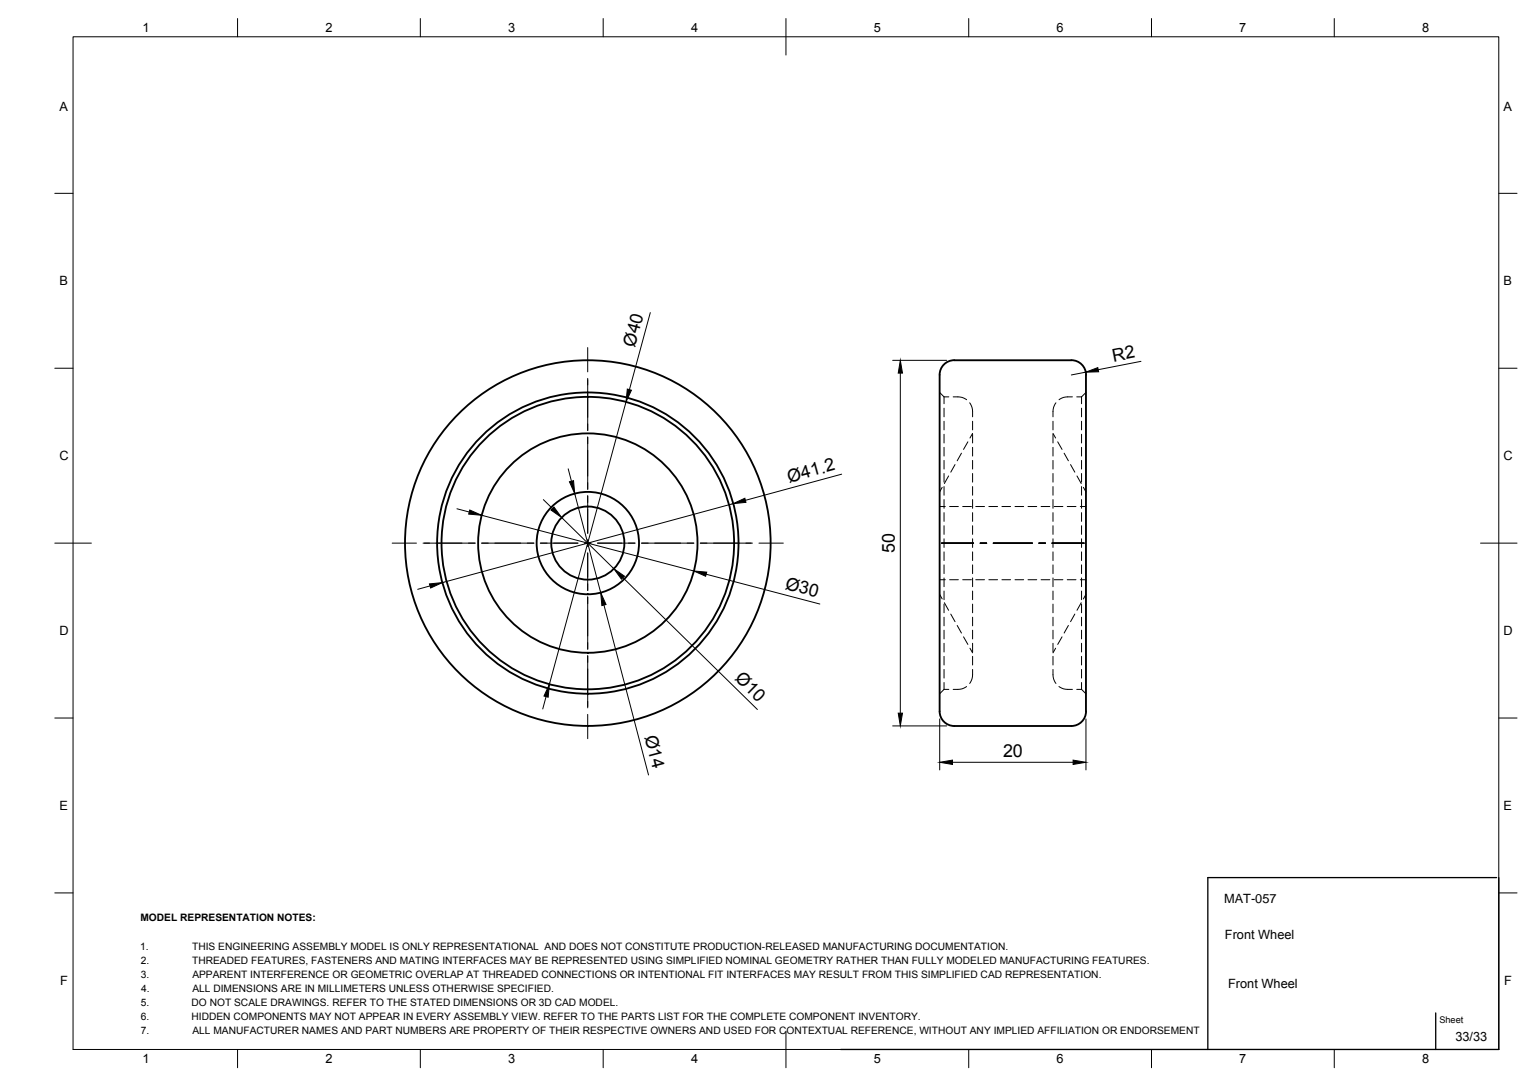
ISO-10303-21;
HEADER;
/* Generated by software containing ST-Developer
 * from STEP Tools, Inc. (www.steptools.com) 
 */

FILE_DESCRIPTION(
/* description */ ('STEP AP214', 'CAx-IF Rec.Pracs.---Representation and Presentation of Product Manufa
cturing Information (PMI)---4.0---2014-10-13'),
/* implementation_level */ '2;1');

FILE_NAME(
/* name */ 'Front Wheel.step',
/* time_stamp */ '2026-10-28T23:34:22+01:00',
/* author */ (''),
/* organization */ (''),
/* preprocessor_version */ 'ST-DEVELOPER v20.2',
/* originating_system */ 'Autodesk Translation Framework v15.17.0.0',
/* authorisation */ '');

FILE_SCHEMA (('AP242_MANAGED_MODEL_BASED_3D_ENGINEERING_MIM_LF { 1 0 10303 442 2 1 4 }'));
ENDSEC;

DATA;
#10=MECHANICAL_DESIGN_GEOMETRIC_PRESENTATION_REPRESENTATION('',(#272),#27807);
#224=SHAPE_REPRESENTATION_RELATIONSHIP('SRR','None',#27923,#246);
#246=ADVANCED_BREP_SHAPE_REPRESENTATION('',(#301),#27803);
#272=STYLED_ITEM('',(#28070),#301);
#301=MANIFOLD_SOLID_BREP('Body1',#12048);
#427=FACE_BOUND('',#2600,.T.);
#428=FACE_BOUND('',#2602,.T.);
#429=FACE_BOUND('',#2604,.T.);
#430=FACE_BOUND('',#2606,.T.);
#431=FACE_BOUND('',#2608,.T.);
#432=FACE_BOUND('',#2610,.T.);
#695=PLANE('',#13506);
#696=PLANE('',#13507);
#697=PLANE('',#13508);
#698=PLANE('',#13509);
#699=PLANE('',#13510);
#700=PLANE('',#13511);
#842=TOROIDAL_SURFACE('',#13475,23.,2.);
#843=TOROIDAL_SURFACE('',#13480,18.,2.);
#844=TOROIDAL_SURFACE('',#13484,23.,2.);
#845=TOROIDAL_SURFACE('',#13489,18.,2.);
#1180=CYLINDRICAL_SURFACE('',#13494,5.00000000000002);
#1181=CYLINDRICAL_SURFACE('',#13500,20.);
#1182=CYLINDRICAL_SURFACE('',#13504,20.);
#1183=CYLINDRICAL_SURFACE('',#13505,25.);
#1798=FACE_OUTER_BOUND('',#2587,.T.);
#1799=FACE_OUTER_BOUND('',#2588,.T.);
#1800=FACE_OUTER_BOUND('',#2589,.T.);
#1801=FACE_OUTER_BOUND('',#2590,.T.);
#1802=FACE_OUTER_BOUND('',#2591,.T.);
#1803=FACE_OUTER_BOUND('',#2592,.T.);
#1804=FACE_OUTER_BOUND('',#2593,.T.);
#1805=FACE_OUTER_BOUND('',#2594,.T.);
#1806=FACE_OUTER_BOUND('',#2595,.T.);
#1807=FACE_OUTER_BOUND('',#2596,.T.);
#1808=FACE_OUTER_BOUND('',#2597,.T.);
#1809=FACE_OUTER_BOUND('',#2598,.T.);
#1810=FACE_OUTER_BOUND('',#2599,.T.);
#1811=FACE_OUTER_BOUND('',#2601,.T.);
#1812=FACE_OUTER_BOUND('',#2603,.T.);
#1813=FACE_OUTER_BOUND('',#2605,.T.);
#1814=FACE_OUTER_BOUND('',#2607,.T.);
#1815=FACE_OUTER_BOUND('',#2609,.T.);
#2587=EDGE_LOOP('',(#10579,#10580,#10581,#10582,#10583));
#2588=EDGE_LOOP('',(#10584,#10585,#10586,#10587));
#2589=EDGE_LOOP('',(#10588,#10589,#10590,#10591,#10592));
#2590=EDGE_LOOP('',(#10593,#10594,#10595,#10596));
#2591=EDGE_LOOP('',(#10597,#10598,#10599,#10600,#10601));
#2592=EDGE_LOOP('',(#10602,#10603,#10604,#10605,#10606));
#2593=EDGE_LOOP('',(#10607,#10608,#10609,#10610));
#2594=EDGE_LOOP('',(#10611,#10612,#10613,#10614));
#2595=EDGE_LOOP('',(#10615,#10616,#10617,#10618));
#2596=EDGE_LOOP('',(#10619,#10620,#10621,#10622));
#2597=EDGE_LOOP('',(#10623,#10624,#10625,#10626,#10627,#10628));
#2598=EDGE_LOOP('',(#10629,#10630,#10631,#10632,#10633,#10634));
#2599=EDGE_LOOP('',(#10635));
#2600=EDGE_LOOP('',(#10636));
#2601=EDGE_LOOP('',(#10637));
#2602=EDGE_LOOP('',(#10638));
#2603=EDGE_LOOP('',(#10639));
#2604=EDGE_LOOP('',(#10640));
#2605=EDGE_LOOP('',(#10641));
#2606=EDGE_LOOP('',(#10642));
#2607=EDGE_LOOP('',(#10643));
#2608=EDGE_LOOP('',(#10644));
#2609=EDGE_LOOP('',(#10645));
#2610=EDGE_LOOP('',(#10646));
#3425=LINE('',#23241,#4245);
#3426=LINE('',#23247,#4246);
#3427=LINE('',#23283,#4247);
#3428=LINE('',#23289,#4248);
#3429=LINE('',#23292,#4249);
#3430=LINE('',#23297,#4250);
#3431=LINE('',#23300,#4251);
#3432=LINE('',#23302,#4252);
#4245=VECTOR('',#16749,20.6);
#4246=VECTOR('',#16756,20.);
#4247=VECTOR('',#16801,5.00000000000002);
#4248=VECTOR('',#16808,7.00000000000002);
#4249=VECTOR('',#16813,20.);
#4250=VECTOR('',#16818,15.);
#4251=VECTOR('',#16823,20.);
#4252=VECTOR('',#16826,25.);
#4940=CIRCLE('',#13469,20.);
#4941=CIRCLE('',#13470,20.);
#4942=CIRCLE('',#13471,20.6);
#4943=CIRCLE('',#13473,20.);
#4944=CIRCLE('',#13474,20.6);
#4945=CIRCLE('',#13476,23.);
#4946=CIRCLE('',#13477,2.);
#4947=CIRCLE('',#13478,25.);
#4948=CIRCLE('',#13479,25.);
#4949=CIRCLE('',#13481,18.);
#4950=CIRCLE('',#13482,2.);
#4951=CIRCLE('',#13483,20.);
#4952=CIRCLE('',#13485,25.);
#4953=CIRCLE('',#13486,25.);
#4954=CIRCLE('',#13487,2.);
#4955=CIRCLE('',#13488,23.);
#4956=CIRCLE('',#13490,18.);
#4957=CIRCLE('',#13491,2.);
#4958=CIRCLE('',#13492,20.);
#4959=CIRCLE('',#13493,20.);
#4960=CIRCLE('',#13495,4.99999999999998);
#4961=CIRCLE('',#13496,5.00000000000002);
#4962=CIRCLE('',#13498,15.);
#4963=CIRCLE('',#13499,7.00000000000002);
#4964=CIRCLE('',#13502,15.);
#4965=CIRCLE('',#13503,7.00000000000002);
#5910=VERTEX_POINT('',#23236);
#5911=VERTEX_POINT('',#23237);
#5912=VERTEX_POINT('',#23240);
#5913=VERTEX_POINT('',#23244);
#5914=VERTEX_POINT('',#23246);
#5915=VERTEX_POINT('',#23250);
#5916=VERTEX_POINT('',#23252);
#5917=VERTEX_POINT('',#23254);
#5918=VERTEX_POINT('',#23258);
#5919=VERTEX_POINT('',#23260);
#5920=VERTEX_POINT('',#23264);
#5921=VERTEX_POINT('',#23265);
#5922=VERTEX_POINT('',#23268);
#5923=VERTEX_POINT('',#23272);
#5924=VERTEX_POINT('',#23274);
#5925=VERTEX_POINT('',#23276);
#5926=VERTEX_POINT('',#23280);
#5927=VERTEX_POINT('',#23282);
#5928=VERTEX_POINT('',#23286);
#5929=VERTEX_POINT('',#23288);
#5930=VERTEX_POINT('',#23294);
#5931=VERTEX_POINT('',#23296);
#7502=EDGE_CURVE('',#5910,#5911,#4940,.T.);
#7503=EDGE_CURVE('',#5911,#5910,#4941,.T.);
#7504=EDGE_CURVE('',#5911,#5912,#3425,.T.);
#7505=EDGE_CURVE('',#5912,#5912,#4942,.T.);
#7506=EDGE_CURVE('',#5913,#5913,#4943,.T.);
#7507=EDGE_CURVE('',#5913,#5914,#3426,.T.);
#7508=EDGE_CURVE('',#5914,#5914,#4944,.T.);
#7509=EDGE_CURVE('',#5915,#5915,#4945,.T.);
#7510=EDGE_CURVE('',#5915,#5916,#4946,.T.);
#7511=EDGE_CURVE('',#5917,#5916,#4947,.T.);
#7512=EDGE_CURVE('',#5916,#5917,#4948,.T.);
#7513=EDGE_CURVE('',#5918,#5918,#4949,.T.);
#7514=EDGE_CURVE('',#5918,#5919,#4950,.T.);
#7515=EDGE_CURVE('',#5919,#5919,#4951,.T.);
#7516=EDGE_CURVE('',#5920,#5921,#4952,.T.);
#7517=EDGE_CURVE('',#5921,#5920,#4953,.T.);
#7518=EDGE_CURVE('',#5921,#5922,#4954,.T.);
#7519=EDGE_CURVE('',#5922,#5922,#4955,.T.);
#7520=EDGE_CURVE('',#5923,#5923,#4956,.T.);
#7521=EDGE_CURVE('',#5923,#5924,#4957,.T.);
#7522=EDGE_CURVE('',#5925,#5924,#4958,.T.);
#7523=EDGE_CURVE('',#5924,#5925,#4959,.T.);
#7524=EDGE_CURVE('',#5926,#5926,#4960,.T.);
#7525=EDGE_CURVE('',#5926,#5927,#3427,.T.);
#7526=EDGE_CURVE('',#5927,#5927,#4961,.T.);
#7527=EDGE_CURVE('',#5928,#5928,#4962,.T.);
#7528=EDGE_CURVE('',#5928,#5929,#3428,.T.);
#7529=EDGE_CURVE('',#5929,#5929,#4963,.T.);
#7530=EDGE_CURVE('',#5919,#5913,#3429,.T.);
#7531=EDGE_CURVE('',#5930,#5930,#4964,.T.);
#7532=EDGE_CURVE('',#5930,#5931,#3430,.T.);
#7533=EDGE_CURVE('',#5931,#5931,#4965,.T.);
#7534=EDGE_CURVE('',#5910,#5925,#3431,.T.);
#7535=EDGE_CURVE('',#5920,#5917,#3432,.T.);
#10579=ORIENTED_EDGE('',*,*,#7502,.F.);
#10580=ORIENTED_EDGE('',*,*,#7503,.F.);
#10581=ORIENTED_EDGE('',*,*,#7504,.T.);
#10582=ORIENTED_EDGE('',*,*,#7505,.F.);
#10583=ORIENTED_EDGE('',*,*,#7504,.F.);
#10584=ORIENTED_EDGE('',*,*,#7506,.F.);
#10585=ORIENTED_EDGE('',*,*,#7507,.T.);
#10586=ORIENTED_EDGE('',*,*,#7508,.F.);
#10587=ORIENTED_EDGE('',*,*,#7507,.F.);
#10588=ORIENTED_EDGE('',*,*,#7509,.F.);
#10589=ORIENTED_EDGE('',*,*,#7510,.T.);
#10590=ORIENTED_EDGE('',*,*,#7511,.F.);
#10591=ORIENTED_EDGE('',*,*,#7512,.F.);
#10592=ORIENTED_EDGE('',*,*,#7510,.F.);
#10593=ORIENTED_EDGE('',*,*,#7513,.F.);
#10594=ORIENTED_EDGE('',*,*,#7514,.T.);
#10595=ORIENTED_EDGE('',*,*,#7515,.F.);
#10596=ORIENTED_EDGE('',*,*,#7514,.F.);
#10597=ORIENTED_EDGE('',*,*,#7516,.F.);
#10598=ORIENTED_EDGE('',*,*,#7517,.F.);
#10599=ORIENTED_EDGE('',*,*,#7518,.T.);
#10600=ORIENTED_EDGE('',*,*,#7519,.F.);
#10601=ORIENTED_EDGE('',*,*,#7518,.F.);
#10602=ORIENTED_EDGE('',*,*,#7520,.F.);
#10603=ORIENTED_EDGE('',*,*,#7521,.T.);
#10604=ORIENTED_EDGE('',*,*,#7522,.F.);
#10605=ORIENTED_EDGE('',*,*,#7523,.F.);
#10606=ORIENTED_EDGE('',*,*,#7521,.F.);
#10607=ORIENTED_EDGE('',*,*,#7524,.T.);
#10608=ORIENTED_EDGE('',*,*,#7525,.T.);
#10609=ORIENTED_EDGE('',*,*,#7526,.T.);
#10610=ORIENTED_EDGE('',*,*,#7525,.F.);
#10611=ORIENTED_EDGE('',*,*,#7527,.T.);
#10612=ORIENTED_EDGE('',*,*,#7528,.T.);
#10613=ORIENTED_EDGE('',*,*,#7529,.F.);
#10614=ORIENTED_EDGE('',*,*,#7528,.F.);
#10615=ORIENTED_EDGE('',*,*,#7515,.T.);
#10616=ORIENTED_EDGE('',*,*,#7530,.T.);
#10617=ORIENTED_EDGE('',*,*,#7506,.T.);
#10618=ORIENTED_EDGE('',*,*,#7530,.F.);
#10619=ORIENTED_EDGE('',*,*,#7531,.F.);
#10620=ORIENTED_EDGE('',*,*,#7532,.T.);
#10621=ORIENTED_EDGE('',*,*,#7533,.T.);
#10622=ORIENTED_EDGE('',*,*,#7532,.F.);
#10623=ORIENTED_EDGE('',*,*,#7502,.T.);
#10624=ORIENTED_EDGE('',*,*,#7503,.T.);
#10625=ORIENTED_EDGE('',*,*,#7534,.T.);
#10626=ORIENTED_EDGE('',*,*,#7522,.T.);
#10627=ORIENTED_EDGE('',*,*,#7523,.T.);
#10628=ORIENTED_EDGE('',*,*,#7534,.F.);
#10629=ORIENTED_EDGE('',*,*,#7516,.T.);
#10630=ORIENTED_EDGE('',*,*,#7517,.T.);
#10631=ORIENTED_EDGE('',*,*,#7535,.T.);
#10632=ORIENTED_EDGE('',*,*,#7511,.T.);
#10633=ORIENTED_EDGE('',*,*,#7512,.T.);
#10634=ORIENTED_EDGE('',*,*,#7535,.F.);
#10635=ORIENTED_EDGE('',*,*,#7509,.T.);
#10636=ORIENTED_EDGE('',*,*,#7508,.T.);
#10637=ORIENTED_EDGE('',*,*,#7519,.T.);
#10638=ORIENTED_EDGE('',*,*,#7505,.T.);
#10639=ORIENTED_EDGE('',*,*,#7520,.T.);
#10640=ORIENTED_EDGE('',*,*,#7531,.T.);
#10641=ORIENTED_EDGE('',*,*,#7513,.T.);
#10642=ORIENTED_EDGE('',*,*,#7527,.F.);
#10643=ORIENTED_EDGE('',*,*,#7533,.F.);
#10644=ORIENTED_EDGE('',*,*,#7524,.F.);
#10645=ORIENTED_EDGE('',*,*,#7529,.T.);
#10646=ORIENTED_EDGE('',*,*,#7526,.F.);
#11314=CONICAL_SURFACE('',#13468,20.6,0.785398163397443);
#11315=CONICAL_SURFACE('',#13472,20.,0.785398163397457);
#11316=CONICAL_SURFACE('',#13497,7.00000000000002,1.05840686648416);
#11317=CONICAL_SURFACE('',#13501,15.,1.05840686648416);
#11880=ADVANCED_FACE('',(#1798),#11314,.F.);
#11881=ADVANCED_FACE('',(#1799),#11315,.F.);
#11882=ADVANCED_FACE('',(#1800),#842,.T.);
#11883=ADVANCED_FACE('',(#1801),#843,.F.);
#11884=ADVANCED_FACE('',(#1802),#844,.T.);
#11885=ADVANCED_FACE('',(#1803),#845,.F.);
#11886=ADVANCED_FACE('',(#1804),#1180,.F.);
#11887=ADVANCED_FACE('',(#1805),#11316,.T.);
#11888=ADVANCED_FACE('',(#1806),#1181,.F.);
#11889=ADVANCED_FACE('',(#1807),#11317,.T.);
#11890=ADVANCED_FACE('',(#1808),#1182,.F.);
#11891=ADVANCED_FACE('',(#1809),#1183,.T.);
#11892=ADVANCED_FACE('',(#1810,#427),#695,.T.);
#11893=ADVANCED_FACE('',(#1811,#428),#696,.F.);
#11894=ADVANCED_FACE('',(#1812,#429),#697,.T.);
#11895=ADVANCED_FACE('',(#1813,#430),#698,.T.);
#11896=ADVANCED_FACE('',(#1814,#431),#699,.F.);
#11897=ADVANCED_FACE('',(#1815,#432),#700,.T.);
#12048=CLOSED_SHELL('',(#11880,#11881,#11882,#11883,#11884,#11885,#11886,
#11887,#11888,#11889,#11890,#11891,#11892,#11893,#11894,#11895,#11896,#11897));
#13467=AXIS2_PLACEMENT_3D('',#23234,#16741,#16742);
#13468=AXIS2_PLACEMENT_3D('',#23235,#16743,#16744);
#13469=AXIS2_PLACEMENT_3D('',#23238,#16745,#16746);
#13470=AXIS2_PLACEMENT_3D('',#23239,#16747,#16748);
#13471=AXIS2_PLACEMENT_3D('',#23242,#16750,#16751);
#13472=AXIS2_PLACEMENT_3D('',#23243,#16752,#16753);
#13473=AXIS2_PLACEMENT_3D('',#23245,#16754,#16755);
#13474=AXIS2_PLACEMENT_3D('',#23248,#16757,#16758);
#13475=AXIS2_PLACEMENT_3D('',#23249,#16759,#16760);
#13476=AXIS2_PLACEMENT_3D('',#23251,#16761,#16762);
#13477=AXIS2_PLACEMENT_3D('',#23253,#16763,#16764);
#13478=AXIS2_PLACEMENT_3D('',#23255,#16765,#16766);
#13479=AXIS2_PLACEMENT_3D('',#23256,#16767,#16768);
#13480=AXIS2_PLACEMENT_3D('',#23257,#16769,#16770);
#13481=AXIS2_PLACEMENT_3D('',#23259,#16771,#16772);
#13482=AXIS2_PLACEMENT_3D('',#23261,#16773,#16774);
#13483=AXIS2_PLACEMENT_3D('',#23262,#16775,#16776);
#13484=AXIS2_PLACEMENT_3D('',#23263,#16777,#16778);
#13485=AXIS2_PLACEMENT_3D('',#23266,#16779,#16780);
#13486=AXIS2_PLACEMENT_3D('',#23267,#16781,#16782);
#13487=AXIS2_PLACEMENT_3D('',#23269,#16783,#16784);
#13488=AXIS2_PLACEMENT_3D('',#23270,#16785,#16786);
#13489=AXIS2_PLACEMENT_3D('',#23271,#16787,#16788);
#13490=AXIS2_PLACEMENT_3D('',#23273,#16789,#16790);
#13491=AXIS2_PLACEMENT_3D('',#23275,#16791,#16792);
#13492=AXIS2_PLACEMENT_3D('',#23277,#16793,#16794);
#13493=AXIS2_PLACEMENT_3D('',#23278,#16795,#16796);
#13494=AXIS2_PLACEMENT_3D('',#23279,#16797,#16798);
#13495=AXIS2_PLACEMENT_3D('',#23281,#16799,#16800);
#13496=AXIS2_PLACEMENT_3D('',#23284,#16802,#16803);
#13497=AXIS2_PLACEMENT_3D('',#23285,#16804,#16805);
#13498=AXIS2_PLACEMENT_3D('',#23287,#16806,#16807);
#13499=AXIS2_PLACEMENT_3D('',#23290,#16809,#16810);
#13500=AXIS2_PLACEMENT_3D('',#23291,#16811,#16812);
#13501=AXIS2_PLACEMENT_3D('',#23293,#16814,#16815);
#13502=AXIS2_PLACEMENT_3D('',#23295,#16816,#16817);
#13503=AXIS2_PLACEMENT_3D('',#23298,#16819,#16820);
#13504=AXIS2_PLACEMENT_3D('',#23299,#16821,#16822);
#13505=AXIS2_PLACEMENT_3D('',#23301,#16824,#16825);
#13506=AXIS2_PLACEMENT_3D('',#23303,#16827,#16828);
#13507=AXIS2_PLACEMENT_3D('',#23304,#16829,#16830);
#13508=AXIS2_PLACEMENT_3D('',#23305,#16831,#16832);
#13509=AXIS2_PLACEMENT_3D('',#23306,#16833,#16834);
#13510=AXIS2_PLACEMENT_3D('',#23307,#16835,#16836);
#13511=AXIS2_PLACEMENT_3D('',#23308,#16837,#16838);
#16741=DIRECTION('axis',(0.,0.,1.));
#16742=DIRECTION('refdir',(1.,0.,0.));
#16743=DIRECTION('center_axis',(0.,0.,1.));
#16744=DIRECTION('ref_axis',(0.916331447796931,0.400420626065117,0.));
#16745=DIRECTION('center_axis',(0.,0.,1.));
#16746=DIRECTION('ref_axis',(-0.916331447796931,-0.400420626065117,0.));
#16747=DIRECTION('center_axis',(0.,0.,1.));
#16748=DIRECTION('ref_axis',(-0.916331447796931,-0.400420626065117,0.));
#16749=DIRECTION('',(-0.647944180551693,-0.283140140017605,0.707106781186552));
#16750=DIRECTION('center_axis',(0.,0.,-1.));
#16751=DIRECTION('ref_axis',(-0.916331447796931,-0.400420626065117,0.));
#16752=DIRECTION('center_axis',(0.,0.,-1.));
#16753=DIRECTION('ref_axis',(-0.916331447796931,-0.400420626065117,0.));
#16754=DIRECTION('center_axis',(0.,0.,-1.));
#16755=DIRECTION('ref_axis',(-0.916331447796931,-0.400420626065117,0.));
#16756=DIRECTION('',(0.647944180551702,0.28314014001761,-0.707106781186541));
#16757=DIRECTION('center_axis',(0.,0.,1.));
#16758=DIRECTION('ref_axis',(-0.916331447796931,-0.400420626065117,0.));
#16759=DIRECTION('center_axis',(0.,0.,-1.));
#16760=DIRECTION('ref_axis',(-0.916331447796931,-0.400420626065117,0.));
#16761=DIRECTION('center_axis',(0.,0.,-1.));
#16762=DIRECTION('ref_axis',(-0.916331447796931,-0.400420626065116,0.));
#16763=DIRECTION('center_axis',(0.400420626065116,-0.916331447796931,0.));
#16764=DIRECTION('ref_axis',(0.916331447796931,0.400420626065116,0.));
#16765=DIRECTION('center_axis',(0.,0.,1.));
#16766=DIRECTION('ref_axis',(-0.916331447796931,-0.400420626065117,0.));
#16767=DIRECTION('center_axis',(0.,0.,1.));
#16768=DIRECTION('ref_axis',(-0.916331447796931,-0.400420626065117,0.));
#16769=DIRECTION('center_axis',(0.,0.,-1.));
#16770=DIRECTION('ref_axis',(-0.916331447796931,-0.400420626065118,0.));
#16771=DIRECTION('center_axis',(0.,0.,-1.));
#16772=DIRECTION('ref_axis',(-0.916331447796931,-0.400420626065117,0.));
#16773=DIRECTION('center_axis',(-0.400420626065117,0.916331447796931,0.));
#16774=DIRECTION('ref_axis',(0.916331447796931,0.400420626065117,0.));
#16775=DIRECTION('center_axis',(0.,0.,1.));
#16776=DIRECTION('ref_axis',(-0.916331447796931,-0.400420626065117,0.));
#16777=DIRECTION('center_axis',(0.,0.,-1.));
#16778=DIRECTION('ref_axis',(-0.916331447796931,-0.400420626065117,0.));
#16779=DIRECTION('center_axis',(0.,0.,-1.));
#16780=DIRECTION('ref_axis',(-0.916331447796931,-0.400420626065117,0.));
#16781=DIRECTION('center_axis',(0.,0.,-1.));
#16782=DIRECTION('ref_axis',(-0.916331447796931,-0.400420626065117,0.));
#16783=DIRECTION('center_axis',(0.400420626065116,-0.916331447796931,0.));
#16784=DIRECTION('ref_axis',(0.916331447796931,0.400420626065116,0.));
#16785=DIRECTION('center_axis',(0.,0.,1.));
#16786=DIRECTION('ref_axis',(-0.916331447796931,-0.400420626065116,0.));
#16787=DIRECTION('center_axis',(0.,0.,1.));
#16788=DIRECTION('ref_axis',(0.916331447796931,0.400420626065118,0.));
#16789=DIRECTION('center_axis',(0.,0.,1.));
#16790=DIRECTION('ref_axis',(0.916331447796931,0.400420626065117,0.));
#16791=DIRECTION('center_axis',(-0.400420626065117,0.916331447796931,0.));
#16792=DIRECTION('ref_axis',(-0.916331447796931,-0.400420626065117,0.));
#16793=DIRECTION('center_axis',(0.,0.,-1.));
#16794=DIRECTION('ref_axis',(0.916331447796931,0.400420626065117,0.));
#16795=DIRECTION('center_axis',(0.,0.,-1.));
#16796=DIRECTION('ref_axis',(0.916331447796931,0.400420626065117,0.));
#16797=DIRECTION('center_axis',(0.,0.,-1.));
#16798=DIRECTION('ref_axis',(-0.916331447796932,-0.400420626065115,0.));
#16799=DIRECTION('center_axis',(0.,0.,1.));
#16800=DIRECTION('ref_axis',(-0.916331447796929,-0.400420626065122,0.));
#16801=DIRECTION('',(0.,0.,-1.));
#16802=DIRECTION('center_axis',(0.,0.,-1.));
#16803=DIRECTION('ref_axis',(-0.916331447796932,-0.400420626065115,0.));
#16804=DIRECTION('center_axis',(0.,0.,1.));
#16805=DIRECTION('ref_axis',(0.916331447796932,0.400420626065116,0.));
#16806=DIRECTION('center_axis',(0.,0.,-1.));
#16807=DIRECTION('ref_axis',(-0.916331447796931,-0.400420626065116,0.));
#16808=DIRECTION('',(0.798652073797726,0.348996822238451,-0.490261239632559));
#16809=DIRECTION('center_axis',(0.,0.,-1.));
#16810=DIRECTION('ref_axis',(-0.916331447796932,-0.400420626065116,0.));
#16811=DIRECTION('center_axis',(0.,0.,-1.));
#16812=DIRECTION('ref_axis',(-0.916331447796931,-0.400420626065117,0.));
#16813=DIRECTION('',(0.,0.,-1.));
#16814=DIRECTION('center_axis',(0.,0.,-1.));
#16815=DIRECTION('ref_axis',(-0.916331447796931,-0.400420626065116,0.));
#16816=DIRECTION('center_axis',(0.,0.,-1.));
#16817=DIRECTION('ref_axis',(-0.916331447796931,-0.400420626065116,0.));
#16818=DIRECTION('',(-0.798652073797726,-0.348996822238452,0.490261239632559));
#16819=DIRECTION('center_axis',(0.,0.,-1.));
#16820=DIRECTION('ref_axis',(-0.916331447796932,-0.400420626065116,0.));
#16821=DIRECTION('center_axis',(0.,0.,-1.));
#16822=DIRECTION('ref_axis',(-0.916331447796931,-0.400420626065117,0.));
#16823=DIRECTION('',(0.,0.,-1.));
#16824=DIRECTION('center_axis',(0.,0.,1.));
#16825=DIRECTION('ref_axis',(0.916331447796931,0.400420626065116,0.));
#16826=DIRECTION('',(0.,0.,-1.));
#16827=DIRECTION('center_axis',(0.,0.,-1.));
#16828=DIRECTION('ref_axis',(-0.916331447796931,-0.400420626065117,0.));
#16829=DIRECTION('center_axis',(0.,0.,-1.));
#16830=DIRECTION('ref_axis',(-0.916331447796931,-0.400420626065117,0.));
#16831=DIRECTION('center_axis',(0.,0.,1.));
#16832=DIRECTION('ref_axis',(0.916331447796931,0.400420626065117,0.));
#16833=DIRECTION('center_axis',(0.,0.,-1.));
#16834=DIRECTION('ref_axis',(-0.916331447796931,-0.400420626065117,0.));
#16835=DIRECTION('center_axis',(0.,0.,-1.));
#16836=DIRECTION('ref_axis',(-0.916331447796931,-0.400420626065117,0.));
#16837=DIRECTION('center_axis',(0.,0.,-1.));
#16838=DIRECTION('ref_axis',(-0.916331447796931,-0.400420626065117,0.));
#23234=CARTESIAN_POINT('',(0.,0.,0.));
#23235=CARTESIAN_POINT('Origin',(-276.958747352154,52.7397376070391,327.323593133701));
#23236=CARTESIAN_POINT('',(-258.632118396215,60.7481501283414,326.723593133701));
#23237=CARTESIAN_POINT('',(-295.285376308092,44.7313250857368,326.723593133701));
#23238=CARTESIAN_POINT('Origin',(-276.958747352154,52.7397376070391,326.723593133701));
#23239=CARTESIAN_POINT('Origin',(-276.958747352154,52.7397376070391,326.723593133701));
#23240=CARTESIAN_POINT('',(-295.83517517677,44.4910727100977,327.323593133701));
#23241=CARTESIAN_POINT('',(-295.83517517677,44.4910727100977,327.323593133701));
#23242=CARTESIAN_POINT('Origin',(-276.958747352154,52.7397376070391,327.323593133701));
#23243=CARTESIAN_POINT('Origin',(-276.958747352154,52.7397376070391,307.923593133701));
#23244=CARTESIAN_POINT('',(-258.632118396215,60.7481501283414,307.923593133701));
#23245=CARTESIAN_POINT('Origin',(-276.958747352154,52.7397376070391,307.923593133701));
#23246=CARTESIAN_POINT('',(-258.082319527537,60.9884025039805,307.323593133701));
#23247=CARTESIAN_POINT('',(-258.632118396215,60.7481501283414,307.923593133701));
#23248=CARTESIAN_POINT('Origin',(-276.958747352154,52.7397376070391,307.323593133701));
#23249=CARTESIAN_POINT('Origin',(-276.958747352154,52.7397376070391,309.323593133701));
#23250=CARTESIAN_POINT('',(-255.883124052824,61.9494120065368,307.323593133701));
#23251=CARTESIAN_POINT('Origin',(-276.958747352154,52.7397376070391,307.323593133701));
#23252=CARTESIAN_POINT('',(-254.05046115723,62.750253258667,309.323593133701));
#23253=CARTESIAN_POINT('Origin',(-255.883124052824,61.9494120065368,309.323593133701));
#23254=CARTESIAN_POINT('',(-299.867033547077,42.7292219554112,309.323593133701));
#23255=CARTESIAN_POINT('Origin',(-276.958747352154,52.7397376070391,309.323593133701));
#23256=CARTESIAN_POINT('Origin',(-276.958747352154,52.7397376070391,309.323593133701));
#23257=CARTESIAN_POINT('Origin',(-276.958747352154,52.7397376070391,309.823593133701));
#23258=CARTESIAN_POINT('',(-260.464781291809,59.9473088762112,311.823593133701));
#23259=CARTESIAN_POINT('Origin',(-276.958747352154,52.7397376070391,311.823593133701));
#23260=CARTESIAN_POINT('',(-258.632118396215,60.7481501283415,309.823593133701));
#23261=CARTESIAN_POINT('Origin',(-260.464781291809,59.9473088762112,309.823593133701));
#23262=CARTESIAN_POINT('Origin',(-276.958747352154,52.7397376070391,309.823593133701));
#23263=CARTESIAN_POINT('Origin',(-276.958747352154,52.7397376070391,325.323593133701));
#23264=CARTESIAN_POINT('',(-299.867033547077,42.7292219554112,325.323593133701));
#23265=CARTESIAN_POINT('',(-254.05046115723,62.750253258667,325.323593133701));
#23266=CARTESIAN_POINT('Origin',(-276.958747352154,52.7397376070391,325.323593133701));
#23267=CARTESIAN_POINT('Origin',(-276.958747352154,52.7397376070391,325.323593133701));
#23268=CARTESIAN_POINT('',(-255.883124052824,61.9494120065368,327.323593133701));
#23269=CARTESIAN_POINT('Origin',(-255.883124052824,61.9494120065368,325.323593133701));
#23270=CARTESIAN_POINT('Origin',(-276.958747352154,52.7397376070391,327.323593133701));
#23271=CARTESIAN_POINT('Origin',(-276.958747352154,52.7397376070391,324.823593133701));
#23272=CARTESIAN_POINT('',(-293.452713412498,45.532166337867,322.823593133701));
#23273=CARTESIAN_POINT('Origin',(-276.958747352154,52.7397376070391,322.823593133701));
#23274=CARTESIAN_POINT('',(-295.285376308092,44.7313250857368,324.823593133701));
#23275=CARTESIAN_POINT('Origin',(-293.452713412498,45.532166337867,324.823593133701));
#23276=CARTESIAN_POINT('',(-258.632118396215,60.7481501283414,324.823593133701));
#23277=CARTESIAN_POINT('Origin',(-276.958747352154,52.7397376070391,324.823593133701));
#23278=CARTESIAN_POINT('Origin',(-276.958747352154,52.7397376070391,324.823593133701));
#23279=CARTESIAN_POINT('Origin',(-276.958747352154,52.7397376070391,327.324593133701));
#23280=CARTESIAN_POINT('',(-272.377090113169,54.7418407373647,327.323593133701));
#23281=CARTESIAN_POINT('Origin',(-276.958747352154,52.7397376070391,327.323593133701));
#23282=CARTESIAN_POINT('',(-272.377090113169,54.7418407373647,307.323593133701));
#23283=CARTESIAN_POINT('',(-272.377090113169,54.7418407373647,327.324593133701));
#23284=CARTESIAN_POINT('Origin',(-276.958747352154,52.7397376070391,307.323593133701));
#23285=CARTESIAN_POINT('Origin',(-276.958747352154,52.7397376070391,307.323593133701));
#23286=CARTESIAN_POINT('',(-290.703719069108,46.7334282160624,311.823593133701));
#23287=CARTESIAN_POINT('Origin',(-276.958747352154,52.7397376070391,311.823593133701));
#23288=CARTESIAN_POINT('',(-283.373067486732,49.9367932245833,307.323593133701));
#23289=CARTESIAN_POINT('',(-283.373067486732,49.9367932245833,307.323593133701));
#23290=CARTESIAN_POINT('Origin',(-276.958747352154,52.7397376070391,307.323593133701));
#23291=CARTESIAN_POINT('Origin',(-276.958747352154,52.7397376070391,317.323593133701));
#23292=CARTESIAN_POINT('',(-258.632118396215,60.7481501283414,317.323593133701));
#23293=CARTESIAN_POINT('Origin',(-276.958747352154,52.7397376070391,322.823593133701));
#23294=CARTESIAN_POINT('',(-263.2137756352,58.7460469980159,322.823593133701));
#23295=CARTESIAN_POINT('Origin',(-276.958747352154,52.7397376070391,322.823593133701));
#23296=CARTESIAN_POINT('',(-270.544427217575,55.5426819894949,327.323593133701));
#23297=CARTESIAN_POINT('',(-263.2137756352,58.7460469980159,322.823593133701));
#23298=CARTESIAN_POINT('Origin',(-276.958747352154,52.7397376070391,327.323593133701));
#23299=CARTESIAN_POINT('Origin',(-276.958747352154,52.7397376070391,317.323593133701));
#23300=CARTESIAN_POINT('',(-258.632118396215,60.7481501283414,317.323593133701));
#23301=CARTESIAN_POINT('Origin',(-276.958747352154,52.7397376070391,307.323593133701));
#23302=CARTESIAN_POINT('',(-299.867033547077,42.7292219554112,307.323593133701));
#23303=CARTESIAN_POINT('Origin',(-276.958747352154,52.7397376070391,307.323593133701));
#23304=CARTESIAN_POINT('Origin',(-276.958747352154,52.7397376070391,327.323593133701));
#23305=CARTESIAN_POINT('Origin',(-284.967159873456,71.0663665629777,322.823593133701));
#23306=CARTESIAN_POINT('Origin',(-284.967159873456,71.0663665629777,311.823593133701));
#23307=CARTESIAN_POINT('Origin',(-276.958747352154,52.7397376070391,327.323593133701));
#23308=CARTESIAN_POINT('Origin',(-276.958747352154,52.7397376070391,307.323593133701));
#27774=UNCERTAINTY_MEASURE_WITH_UNIT(LENGTH_MEASURE(0.01),#27808,
'DISTANCE_ACCURACY_VALUE',
'Maximum model space distance between geometric entities at asserted c
onnectivities');
#27778=UNCERTAINTY_MEASURE_WITH_UNIT(LENGTH_MEASURE(0.01),#27808,
'DISTANCE_ACCURACY_VALUE',
'Maximum model space distance between geometric entities at asserted c
onnectivities');
#27803=(
GEOMETRIC_REPRESENTATION_CONTEXT(3)
GLOBAL_UNCERTAINTY_ASSIGNED_CONTEXT((#27774))
GLOBAL_UNIT_ASSIGNED_CONTEXT((#27808,#27810,#27811))
REPRESENTATION_CONTEXT('','3D')
);
#27807=(
GEOMETRIC_REPRESENTATION_CONTEXT(3)
GLOBAL_UNCERTAINTY_ASSIGNED_CONTEXT((#27778))
GLOBAL_UNIT_ASSIGNED_CONTEXT((#27808,#27810,#27811))
REPRESENTATION_CONTEXT('','3D')
);
#27808=(
LENGTH_UNIT()
NAMED_UNIT(*)
SI_UNIT(.MILLI.,.METRE.)
);
#27810=(
NAMED_UNIT(*)
PLANE_ANGLE_UNIT()
SI_UNIT($,.RADIAN.)
);
#27811=(
NAMED_UNIT(*)
SI_UNIT($,.STERADIAN.)
SOLID_ANGLE_UNIT()
);
#27836=SHAPE_DEFINITION_REPRESENTATION(#27879,#27923);
#27879=PRODUCT_DEFINITION_SHAPE('',$,#27952);
#27923=SHAPE_REPRESENTATION('',(#13467),#27803);
#27927=PRODUCT_DEFINITION_CONTEXT('part definition',#28013,'design');
#27952=PRODUCT_DEFINITION('Front Wheel','Front Wheel',#27980,#27927);
#27980=PRODUCT_DEFINITION_FORMATION('',$,#28039);
#28013=APPLICATION_CONTEXT('Managed model based 3d engineering');
#28014=PRODUCT_CONTEXT('part definition',#28013,'mechanical');
#28039=PRODUCT('Front Wheel','Front Wheel',$,(#28014));
#28064=COLOUR_RGB('Sky Blue',0.24,0.69,0.87);
#28065=FILL_AREA_STYLE_COLOUR('',#28064);
#28066=FILL_AREA_STYLE('',(#28065));
#28067=SURFACE_STYLE_FILL_AREA(#28066);
#28068=SURFACE_SIDE_STYLE('',(#28067));
#28069=SURFACE_STYLE_USAGE(.BOTH.,#28068);
#28070=PRESENTATION_STYLE_ASSIGNMENT((#28069));
ENDSEC;
END-ISO-10303-21;
